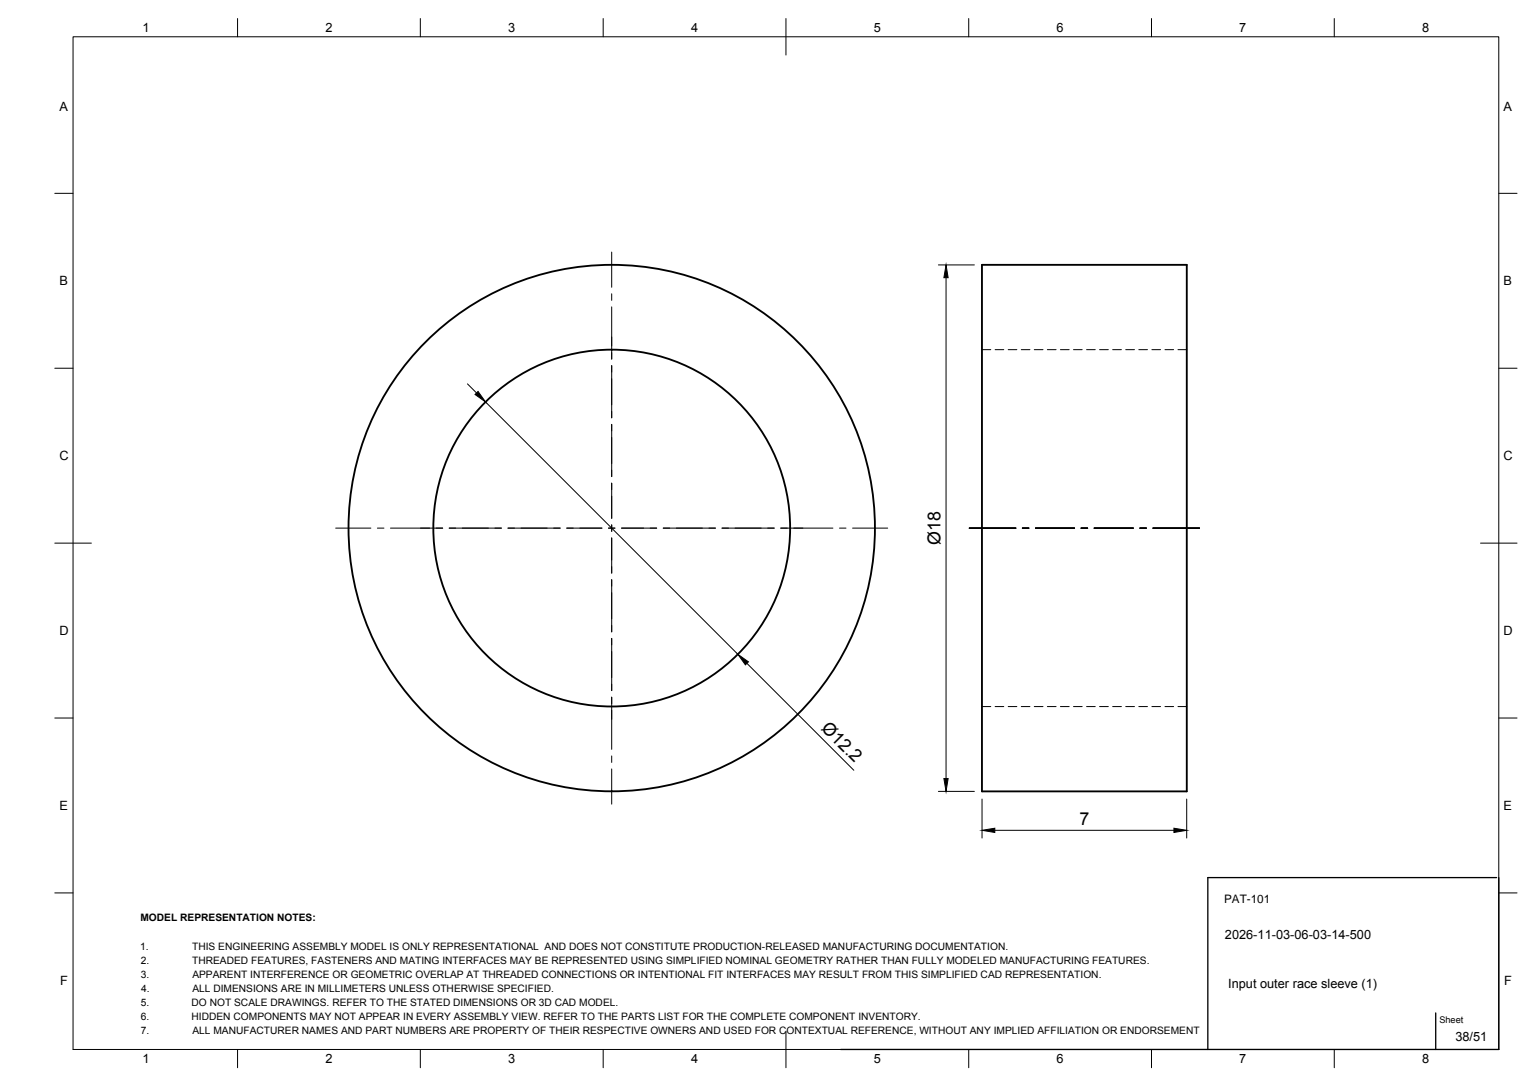
ISO-10303-21;
HEADER;
/* Generated by software containing ST-Developer
 * from STEP Tools, Inc. (www.steptools.com) 
 */

FILE_DESCRIPTION(
/* description */ ('Spur gear reduction stage 2-1 on bearing plates'),
/* implementation_level */ '2;1');

FILE_NAME(
/* name */ 'Input outer race sleeve (1).step',
/* time_stamp */ '2026-10-28T03:22:07-07:00',
/* author */ (''),
/* organization */ (''),
/* preprocessor_version */ 'ST-DEVELOPER v20.2',
/* originating_system */ 'Autodesk Translation Framework v15.17.0.0',
/* authorisation */ '');

FILE_SCHEMA (('AUTOMOTIVE_DESIGN { 1 0 10303 214 3 1 1 }'));
ENDSEC;

DATA;
#10=MECHANICAL_DESIGN_GEOMETRIC_PRESENTATION_REPRESENTATION('',(#992),#53909);
#891=SHAPE_REPRESENTATION_RELATIONSHIP('SRR','None',#54121,#934);
#934=ADVANCED_BREP_SHAPE_REPRESENTATION('',(#1047),#53895);
#992=STYLED_ITEM('',(#54397),#1047);
#1047=MANIFOLD_SOLID_BREP('Body1',#11319);
#1212=FACE_BOUND('',#2620,.T.);
#1213=FACE_BOUND('',#2622,.T.);
#1379=PLANE('',#12558);
#1380=PLANE('',#12559);
#1817=FACE_OUTER_BOUND('',#2617,.T.);
#1818=FACE_OUTER_BOUND('',#2618,.T.);
#1819=FACE_OUTER_BOUND('',#2619,.T.);
#1820=FACE_OUTER_BOUND('',#2621,.T.);
#2617=EDGE_LOOP('',(#8612,#8613,#8614,#8615));
#2618=EDGE_LOOP('',(#8616,#8617,#8618,#8619));
#2619=EDGE_LOOP('',(#8620));
#2620=EDGE_LOOP('',(#8621));
#2621=EDGE_LOOP('',(#8622));
#2622=EDGE_LOOP('',(#8623));
#3220=LINE('',#18178,#3861);
#3221=LINE('',#18184,#3862);
#3861=VECTOR('',#14721,0.61);
#3862=VECTOR('',#14728,0.9);
#4606=CIRCLE('',#12553,0.61);
#4607=CIRCLE('',#12554,0.61);
#4608=CIRCLE('',#12556,0.9);
#4609=CIRCLE('',#12557,0.9);
#5218=VERTEX_POINT('',#18175);
#5219=VERTEX_POINT('',#18177);
#5220=VERTEX_POINT('',#18181);
#5221=VERTEX_POINT('',#18183);
#6448=EDGE_CURVE('',#5218,#5218,#4606,.T.);
#6449=EDGE_CURVE('',#5218,#5219,#3220,.T.);
#6450=EDGE_CURVE('',#5219,#5219,#4607,.T.);
#6451=EDGE_CURVE('',#5220,#5220,#4608,.T.);
#6452=EDGE_CURVE('',#5220,#5221,#3221,.T.);
#6453=EDGE_CURVE('',#5221,#5221,#4609,.T.);
#8612=ORIENTED_EDGE('',*,*,#6448,.F.);
#8613=ORIENTED_EDGE('',*,*,#6449,.T.);
#8614=ORIENTED_EDGE('',*,*,#6450,.T.);
#8615=ORIENTED_EDGE('',*,*,#6449,.F.);
#8616=ORIENTED_EDGE('',*,*,#6451,.F.);
#8617=ORIENTED_EDGE('',*,*,#6452,.T.);
#8618=ORIENTED_EDGE('',*,*,#6453,.T.);
#8619=ORIENTED_EDGE('',*,*,#6452,.F.);
#8620=ORIENTED_EDGE('',*,*,#6451,.T.);
#8621=ORIENTED_EDGE('',*,*,#6448,.T.);
#8622=ORIENTED_EDGE('',*,*,#6453,.F.);
#8623=ORIENTED_EDGE('',*,*,#6450,.F.);
#10539=CYLINDRICAL_SURFACE('',#12552,0.61);
#10540=CYLINDRICAL_SURFACE('',#12555,0.9);
#10937=ADVANCED_FACE('',(#1817),#10539,.F.);
#10938=ADVANCED_FACE('',(#1818),#10540,.T.);
#10939=ADVANCED_FACE('',(#1819,#1212),#1379,.T.);
#10940=ADVANCED_FACE('',(#1820,#1213),#1380,.F.);
#11319=CLOSED_SHELL('',(#10937,#10938,#10939,#10940));
#12551=AXIS2_PLACEMENT_3D('',#18173,#14715,#14716);
#12552=AXIS2_PLACEMENT_3D('',#18174,#14717,#14718);
#12553=AXIS2_PLACEMENT_3D('',#18176,#14719,#14720);
#12554=AXIS2_PLACEMENT_3D('',#18179,#14722,#14723);
#12555=AXIS2_PLACEMENT_3D('',#18180,#14724,#14725);
#12556=AXIS2_PLACEMENT_3D('',#18182,#14726,#14727);
#12557=AXIS2_PLACEMENT_3D('',#18185,#14729,#14730);
#12558=AXIS2_PLACEMENT_3D('',#18186,#14731,#14732);
#12559=AXIS2_PLACEMENT_3D('',#18187,#14733,#14734);
#14715=DIRECTION('axis',(0.,0.,1.));
#14716=DIRECTION('refdir',(1.,0.,0.));
#14717=DIRECTION('center_axis',(0.,1.,0.));
#14718=DIRECTION('ref_axis',(1.,0.,0.));
#14719=DIRECTION('center_axis',(0.,-1.,0.));
#14720=DIRECTION('ref_axis',(1.,0.,0.));
#14721=DIRECTION('',(0.,-1.,0.));
#14722=DIRECTION('center_axis',(0.,-1.,0.));
#14723=DIRECTION('ref_axis',(1.,0.,0.));
#14724=DIRECTION('center_axis',(0.,1.,0.));
#14725=DIRECTION('ref_axis',(1.,0.,0.));
#14726=DIRECTION('center_axis',(0.,1.,0.));
#14727=DIRECTION('ref_axis',(1.,0.,0.));
#14728=DIRECTION('',(0.,-1.,0.));
#14729=DIRECTION('center_axis',(0.,1.,0.));
#14730=DIRECTION('ref_axis',(1.,0.,0.));
#14731=DIRECTION('center_axis',(0.,1.,0.));
#14732=DIRECTION('ref_axis',(1.,0.,0.));
#14733=DIRECTION('center_axis',(0.,1.,0.));
#14734=DIRECTION('ref_axis',(1.,0.,0.));
#18173=CARTESIAN_POINT('',(0.,0.,0.));
#18174=CARTESIAN_POINT('Origin',(0.,4.,0.));
#18175=CARTESIAN_POINT('',(-0.61,4.7,7.47034547479885E-17));
#18176=CARTESIAN_POINT('Origin',(0.,4.7,0.));
#18177=CARTESIAN_POINT('',(-0.61,4.,7.47034547479885E-17));
#18178=CARTESIAN_POINT('',(-0.61,4.,7.47034547479885E-17));
#18179=CARTESIAN_POINT('Origin',(0.,4.,0.));
#18180=CARTESIAN_POINT('Origin',(0.,4.,0.));
#18181=CARTESIAN_POINT('',(-0.9,4.7,1.10218211923262E-16));
#18182=CARTESIAN_POINT('Origin',(0.,4.7,0.));
#18183=CARTESIAN_POINT('',(-0.9,4.,1.10218211923262E-16));
#18184=CARTESIAN_POINT('',(-0.9,4.,1.10218211923262E-16));
#18185=CARTESIAN_POINT('Origin',(0.,4.,0.));
#18186=CARTESIAN_POINT('Origin',(0.,4.7,0.));
#18187=CARTESIAN_POINT('Origin',(0.,4.,0.));
#53845=UNCERTAINTY_MEASURE_WITH_UNIT(LENGTH_MEASURE(0.001),#53910,
'DISTANCE_ACCURACY_VALUE',
'Maximum model space distance between geometric entities at asserted c
onnectivities');
#53859=UNCERTAINTY_MEASURE_WITH_UNIT(LENGTH_MEASURE(0.001),#53910,
'DISTANCE_ACCURACY_VALUE',
'Maximum model space distance between geometric entities at asserted c
onnectivities');
#53895=(
GEOMETRIC_REPRESENTATION_CONTEXT(3)
GLOBAL_UNCERTAINTY_ASSIGNED_CONTEXT((#53845))
GLOBAL_UNIT_ASSIGNED_CONTEXT((#53910,#53912,#53913))
REPRESENTATION_CONTEXT('','3D')
);
#53909=(
GEOMETRIC_REPRESENTATION_CONTEXT(3)
GLOBAL_UNCERTAINTY_ASSIGNED_CONTEXT((#53859))
GLOBAL_UNIT_ASSIGNED_CONTEXT((#53910,#53912,#53913))
REPRESENTATION_CONTEXT('','3D')
);
#53910=(
LENGTH_UNIT()
NAMED_UNIT(*)
SI_UNIT(.CENTI.,.METRE.)
);
#53912=(
NAMED_UNIT(*)
PLANE_ANGLE_UNIT()
SI_UNIT($,.RADIAN.)
);
#53913=(
NAMED_UNIT(*)
SI_UNIT($,.STERADIAN.)
SOLID_ANGLE_UNIT()
);
#53949=SHAPE_DEFINITION_REPRESENTATION(#54047,#54121);
#54047=PRODUCT_DEFINITION_SHAPE('',$,#54171);
#54121=SHAPE_REPRESENTATION('',(#12551),#53895);
#54135=PRODUCT_DEFINITION_CONTEXT('part definition',#54284,'design');
#54171=PRODUCT_DEFINITION('Input outer race sleeve (1)',
'Input outer race sleeve (1)',#54220,#54135);
#54220=PRODUCT_DEFINITION_FORMATION('',$,#54321);
#54284=APPLICATION_CONTEXT(
'Core Data for Automotive Mechanical Design Process');
#54285=PRODUCT_CONTEXT('part definition',#54284,'mechanical');
#54321=PRODUCT('Input outer race sleeve (1)',
'Input outer race sleeve (1)','Input outer race sleeve (1)',(#54285));
#54391=COLOUR_RGB('Grey',0.48,0.52,0.57);
#54392=FILL_AREA_STYLE_COLOUR('',#54391);
#54393=FILL_AREA_STYLE('',(#54392));
#54394=SURFACE_STYLE_FILL_AREA(#54393);
#54395=SURFACE_SIDE_STYLE('',(#54394));
#54396=SURFACE_STYLE_USAGE(.BOTH.,#54395);
#54397=PRESENTATION_STYLE_ASSIGNMENT((#54396));
ENDSEC;
END-ISO-10303-21;
